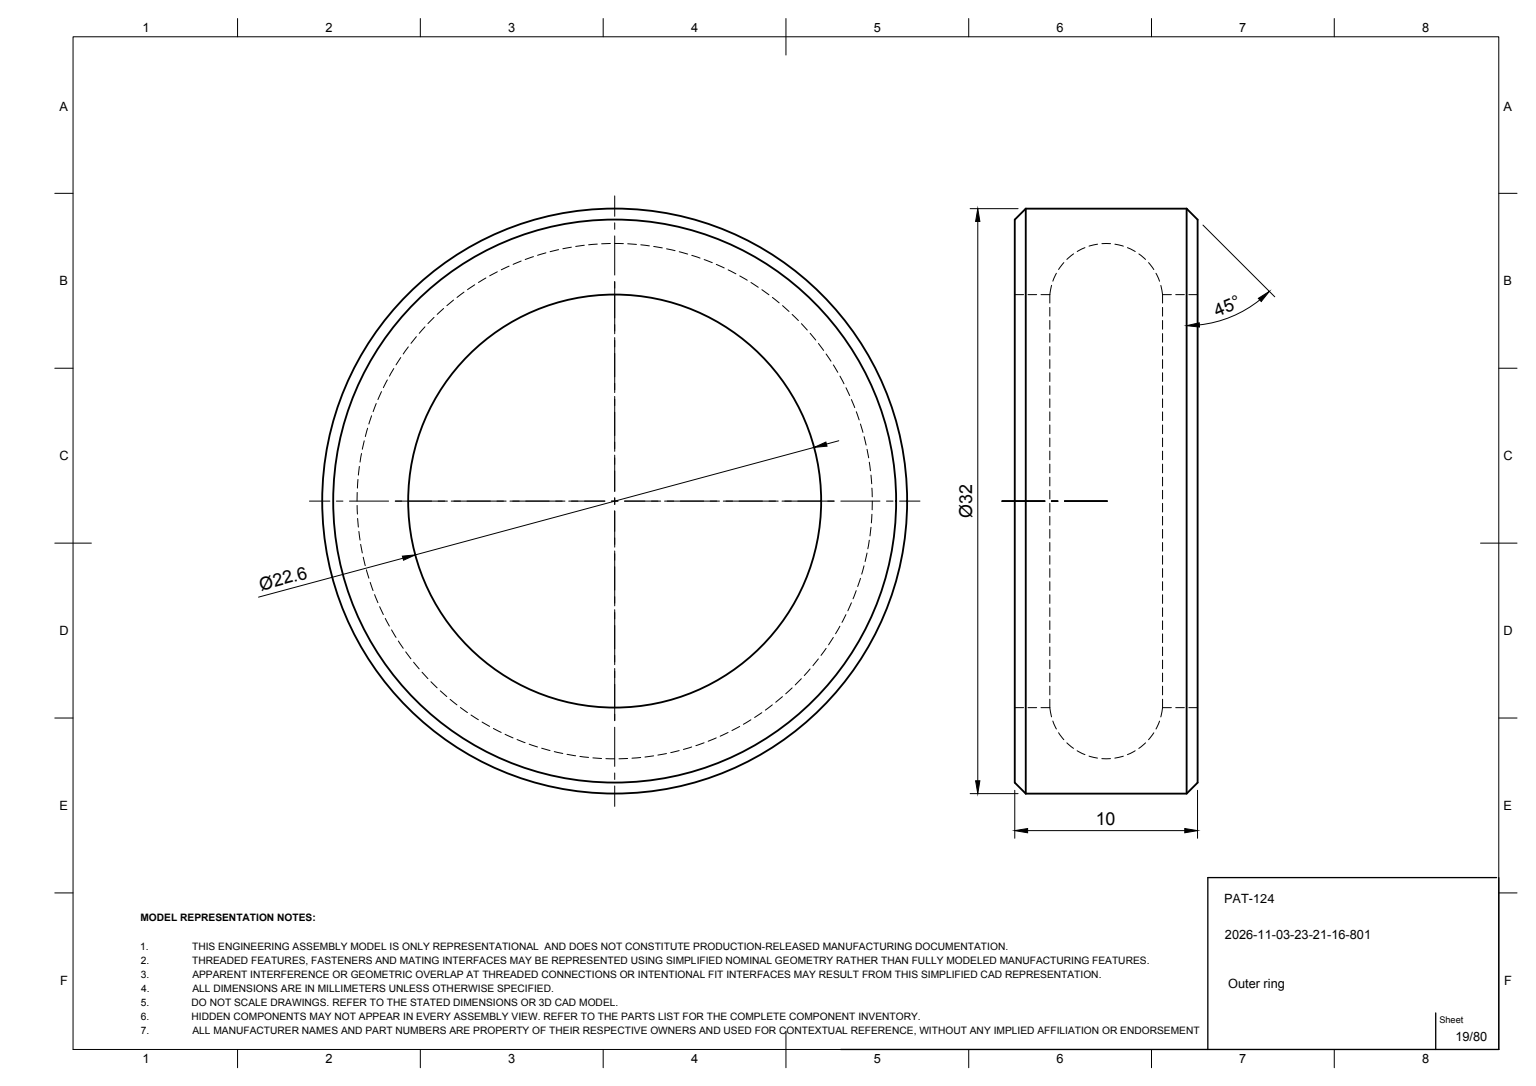
ISO-10303-21;
HEADER;
/* Generated by software containing ST-Developer
 * from STEP Tools, Inc. (www.steptools.com) 
 */

FILE_DESCRIPTION(
/* description */ ('XY cross-slide table'),
/* implementation_level */ '2;1');

FILE_NAME(
/* name */ 'Outer ring.step',
/* time_stamp */ '2026-10-28T03:22:46-07:00',
/* author */ (''),
/* organization */ (''),
/* preprocessor_version */ 'ST-DEVELOPER v20.2',
/* originating_system */ 'Autodesk Translation Framework v15.17.0.0',
/* authorisation */ '');

FILE_SCHEMA (('AUTOMOTIVE_DESIGN { 1 0 10303 214 3 1 1 }'));
ENDSEC;

DATA;
#10=MECHANICAL_DESIGN_GEOMETRIC_PRESENTATION_REPRESENTATION('',(#1682),#62984);
#1443=CONICAL_SURFACE('',#24318,1.57,0.785398163397449);
#1444=CONICAL_SURFACE('',#24322,1.57,0.785398163397449);
#1497=TOROIDAL_SURFACE('',#24307,1.1,0.309556);
#1516=SHAPE_REPRESENTATION_RELATIONSHIP('SRR','None',#63365,#1599);
#1599=ADVANCED_BREP_SHAPE_REPRESENTATION('',(#1795),#62902);
#1682=STYLED_ITEM('',(#63912),#1795);
#1795=MANIFOLD_SOLID_BREP('Body1',#22976);
#1985=FACE_BOUND('',#4439,.T.);
#1986=FACE_BOUND('',#4444,.T.);
#2383=PLANE('',#24315);
#2384=PLANE('',#24324);
#3024=FACE_OUTER_BOUND('',#4436,.T.);
#3025=FACE_OUTER_BOUND('',#4437,.T.);
#3026=FACE_OUTER_BOUND('',#4438,.T.);
#3027=FACE_OUTER_BOUND('',#4440,.T.);
#3028=FACE_OUTER_BOUND('',#4441,.T.);
#3029=FACE_OUTER_BOUND('',#4442,.T.);
#3030=FACE_OUTER_BOUND('',#4443,.T.);
#3031=FACE_OUTER_BOUND('',#4445,.T.);
#4436=EDGE_LOOP('',(#15586,#15587,#15588,#15589,#15590,#15591));
#4437=EDGE_LOOP('',(#15592,#15593,#15594,#15595,#15596));
#4438=EDGE_LOOP('',(#15597));
#4439=EDGE_LOOP('',(#15598));
#4440=EDGE_LOOP('',(#15599,#15600,#15601,#15602));
#4441=EDGE_LOOP('',(#15603,#15604,#15605,#15606));
#4442=EDGE_LOOP('',(#15607,#15608,#15609,#15610));
#4443=EDGE_LOOP('',(#15611));
#4444=EDGE_LOOP('',(#15612));
#4445=EDGE_LOOP('',(#15613,#15614,#15615,#15616,#15617));
#6112=LINE('',#33620,#7599);
#6113=LINE('',#33629,#7600);
#6114=LINE('',#33633,#7601);
#6115=LINE('',#33637,#7602);
#6116=LINE('',#33640,#7603);
#7599=VECTOR('',#27297,1.129765);
#7600=VECTOR('',#27308,1.57);
#7601=VECTOR('',#27313,1.6);
#7602=VECTOR('',#27318,1.57);
#7603=VECTOR('',#27323,1.129765);
#9015=CIRCLE('',#24308,1.129765);
#9016=CIRCLE('',#24309,1.129765);
#9017=CIRCLE('',#24310,0.309556);
#9018=CIRCLE('',#24311,1.129765);
#9019=CIRCLE('',#24312,1.129765);
#9020=CIRCLE('',#24314,1.129765);
#9021=CIRCLE('',#24316,1.54);
#9022=CIRCLE('',#24317,1.129765);
#9023=CIRCLE('',#24319,1.6);
#9024=CIRCLE('',#24321,1.6);
#9025=CIRCLE('',#24323,1.54);
#9997=VERTEX_POINT('',#33608);
#9998=VERTEX_POINT('',#33609);
#9999=VERTEX_POINT('',#33612);
#10000=VERTEX_POINT('',#33614);
#10001=VERTEX_POINT('',#33618);
#10002=VERTEX_POINT('',#33622);
#10003=VERTEX_POINT('',#33624);
#10004=VERTEX_POINT('',#33627);
#10005=VERTEX_POINT('',#33631);
#10006=VERTEX_POINT('',#33635);
#12177=EDGE_CURVE('',#9997,#9998,#9015,.T.);
#12178=EDGE_CURVE('',#9998,#9997,#9016,.T.);
#12179=EDGE_CURVE('',#9998,#9999,#9017,.T.);
#12180=EDGE_CURVE('',#10000,#9999,#9018,.T.);
#12181=EDGE_CURVE('',#9999,#10000,#9019,.T.);
#12182=EDGE_CURVE('',#10001,#10001,#9020,.T.);
#12183=EDGE_CURVE('',#10001,#10000,#6112,.T.);
#12184=EDGE_CURVE('',#10002,#10002,#9021,.T.);
#12185=EDGE_CURVE('',#10003,#10003,#9022,.T.);
#12186=EDGE_CURVE('',#10004,#10004,#9023,.T.);
#12187=EDGE_CURVE('',#10004,#10002,#6113,.T.);
#12188=EDGE_CURVE('',#10005,#10005,#9024,.T.);
#12189=EDGE_CURVE('',#10005,#10004,#6114,.T.);
#12190=EDGE_CURVE('',#10006,#10006,#9025,.T.);
#12191=EDGE_CURVE('',#10006,#10005,#6115,.T.);
#12192=EDGE_CURVE('',#9997,#10003,#6116,.T.);
#15586=ORIENTED_EDGE('',*,*,#12177,.F.);
#15587=ORIENTED_EDGE('',*,*,#12178,.F.);
#15588=ORIENTED_EDGE('',*,*,#12179,.T.);
#15589=ORIENTED_EDGE('',*,*,#12180,.F.);
#15590=ORIENTED_EDGE('',*,*,#12181,.F.);
#15591=ORIENTED_EDGE('',*,*,#12179,.F.);
#15592=ORIENTED_EDGE('',*,*,#12182,.T.);
#15593=ORIENTED_EDGE('',*,*,#12183,.T.);
#15594=ORIENTED_EDGE('',*,*,#12180,.T.);
#15595=ORIENTED_EDGE('',*,*,#12181,.T.);
#15596=ORIENTED_EDGE('',*,*,#12183,.F.);
#15597=ORIENTED_EDGE('',*,*,#12184,.F.);
#15598=ORIENTED_EDGE('',*,*,#12185,.T.);
#15599=ORIENTED_EDGE('',*,*,#12186,.F.);
#15600=ORIENTED_EDGE('',*,*,#12187,.T.);
#15601=ORIENTED_EDGE('',*,*,#12184,.T.);
#15602=ORIENTED_EDGE('',*,*,#12187,.F.);
#15603=ORIENTED_EDGE('',*,*,#12188,.F.);
#15604=ORIENTED_EDGE('',*,*,#12189,.T.);
#15605=ORIENTED_EDGE('',*,*,#12186,.T.);
#15606=ORIENTED_EDGE('',*,*,#12189,.F.);
#15607=ORIENTED_EDGE('',*,*,#12190,.F.);
#15608=ORIENTED_EDGE('',*,*,#12191,.T.);
#15609=ORIENTED_EDGE('',*,*,#12188,.T.);
#15610=ORIENTED_EDGE('',*,*,#12191,.F.);
#15611=ORIENTED_EDGE('',*,*,#12190,.T.);
#15612=ORIENTED_EDGE('',*,*,#12182,.F.);
#15613=ORIENTED_EDGE('',*,*,#12177,.T.);
#15614=ORIENTED_EDGE('',*,*,#12178,.T.);
#15615=ORIENTED_EDGE('',*,*,#12192,.T.);
#15616=ORIENTED_EDGE('',*,*,#12185,.F.);
#15617=ORIENTED_EDGE('',*,*,#12192,.F.);
#21105=CYLINDRICAL_SURFACE('',#24313,1.129765);
#21106=CYLINDRICAL_SURFACE('',#24320,1.6);
#21107=CYLINDRICAL_SURFACE('',#24325,1.129765);
#21805=ADVANCED_FACE('',(#3024),#1497,.F.);
#21806=ADVANCED_FACE('',(#3025),#21105,.F.);
#21807=ADVANCED_FACE('',(#3026,#1985),#2383,.T.);
#21808=ADVANCED_FACE('',(#3027),#1443,.T.);
#21809=ADVANCED_FACE('',(#3028),#21106,.T.);
#21810=ADVANCED_FACE('',(#3029),#1444,.T.);
#21811=ADVANCED_FACE('',(#3030,#1986),#2384,.T.);
#21812=ADVANCED_FACE('',(#3031),#21107,.F.);
#22976=CLOSED_SHELL('',(#21805,#21806,#21807,#21808,#21809,#21810,#21811,
#21812));
#24306=AXIS2_PLACEMENT_3D('',#33606,#27279,#27280);
#24307=AXIS2_PLACEMENT_3D('',#33607,#27281,#27282);
#24308=AXIS2_PLACEMENT_3D('',#33610,#27283,#27284);
#24309=AXIS2_PLACEMENT_3D('',#33611,#27285,#27286);
#24310=AXIS2_PLACEMENT_3D('',#33613,#27287,#27288);
#24311=AXIS2_PLACEMENT_3D('',#33615,#27289,#27290);
#24312=AXIS2_PLACEMENT_3D('',#33616,#27291,#27292);
#24313=AXIS2_PLACEMENT_3D('',#33617,#27293,#27294);
#24314=AXIS2_PLACEMENT_3D('',#33619,#27295,#27296);
#24315=AXIS2_PLACEMENT_3D('',#33621,#27298,#27299);
#24316=AXIS2_PLACEMENT_3D('',#33623,#27300,#27301);
#24317=AXIS2_PLACEMENT_3D('',#33625,#27302,#27303);
#24318=AXIS2_PLACEMENT_3D('',#33626,#27304,#27305);
#24319=AXIS2_PLACEMENT_3D('',#33628,#27306,#27307);
#24320=AXIS2_PLACEMENT_3D('',#33630,#27309,#27310);
#24321=AXIS2_PLACEMENT_3D('',#33632,#27311,#27312);
#24322=AXIS2_PLACEMENT_3D('',#33634,#27314,#27315);
#24323=AXIS2_PLACEMENT_3D('',#33636,#27316,#27317);
#24324=AXIS2_PLACEMENT_3D('',#33638,#27319,#27320);
#24325=AXIS2_PLACEMENT_3D('',#33639,#27321,#27322);
#27279=DIRECTION('axis',(0.,0.,1.));
#27280=DIRECTION('refdir',(1.,0.,0.));
#27281=DIRECTION('center_axis',(0.,-1.,0.));
#27282=DIRECTION('ref_axis',(0.,0.,-1.));
#27283=DIRECTION('center_axis',(0.,-1.,0.));
#27284=DIRECTION('ref_axis',(1.,0.,0.));
#27285=DIRECTION('center_axis',(0.,-1.,0.));
#27286=DIRECTION('ref_axis',(1.,0.,0.));
#27287=DIRECTION('center_axis',(1.,0.,1.22464679914735E-16));
#27288=DIRECTION('ref_axis',(-1.22464679914735E-16,0.,1.));
#27289=DIRECTION('center_axis',(0.,1.,0.));
#27290=DIRECTION('ref_axis',(1.,0.,0.));
#27291=DIRECTION('center_axis',(0.,1.,0.));
#27292=DIRECTION('ref_axis',(1.,0.,0.));
#27293=DIRECTION('center_axis',(0.,-1.,0.));
#27294=DIRECTION('ref_axis',(1.,0.,0.));
#27295=DIRECTION('center_axis',(0.,-1.,0.));
#27296=DIRECTION('ref_axis',(1.,0.,0.));
#27297=DIRECTION('',(0.,1.,0.));
#27298=DIRECTION('center_axis',(0.,1.,0.));
#27299=DIRECTION('ref_axis',(0.,0.,1.));
#27300=DIRECTION('center_axis',(0.,-1.,0.));
#27301=DIRECTION('ref_axis',(1.,0.,0.));
#27302=DIRECTION('center_axis',(0.,-1.,0.));
#27303=DIRECTION('ref_axis',(1.,0.,0.));
#27304=DIRECTION('center_axis',(0.,-1.,0.));
#27305=DIRECTION('ref_axis',(1.,0.,0.));
#27306=DIRECTION('center_axis',(0.,-1.,0.));
#27307=DIRECTION('ref_axis',(1.,0.,0.));
#27308=DIRECTION('',(0.707106781186548,0.707106781186547,8.65956056235494E-17));
#27309=DIRECTION('center_axis',(0.,-1.,0.));
#27310=DIRECTION('ref_axis',(1.,0.,0.));
#27311=DIRECTION('center_axis',(0.,-1.,0.));
#27312=DIRECTION('ref_axis',(1.,0.,0.));
#27313=DIRECTION('',(0.,1.,0.));
#27314=DIRECTION('center_axis',(0.,1.,0.));
#27315=DIRECTION('ref_axis',(1.,0.,0.));
#27316=DIRECTION('center_axis',(0.,-1.,0.));
#27317=DIRECTION('ref_axis',(1.,0.,0.));
#27318=DIRECTION('',(-0.707106781186548,0.707106781186547,-8.65956056235494E-17));
#27319=DIRECTION('center_axis',(0.,-1.,0.));
#27320=DIRECTION('ref_axis',(0.,0.,-1.));
#27321=DIRECTION('center_axis',(0.,-1.,0.));
#27322=DIRECTION('ref_axis',(1.,0.,0.));
#27323=DIRECTION('',(0.,1.,0.));
#33606=CARTESIAN_POINT('',(0.,0.,0.));
#33607=CARTESIAN_POINT('Origin',(0.,0.,0.));
#33608=CARTESIAN_POINT('',(-1.129765,0.308121667383195,-1.38356309103871E-16));
#33609=CARTESIAN_POINT('',(-1.38356309103871E-16,0.308121667383195,1.129765));
#33610=CARTESIAN_POINT('Origin',(0.,0.308121667383195,0.));
#33611=CARTESIAN_POINT('Origin',(0.,0.308121667383195,0.));
#33612=CARTESIAN_POINT('',(-1.38356309103871E-16,-0.308121667383195,1.129765));
#33613=CARTESIAN_POINT('Origin',(-1.34711147906209E-16,0.,1.1));
#33614=CARTESIAN_POINT('',(-1.129765,-0.308121667383195,1.38356309103871E-16));
#33615=CARTESIAN_POINT('Origin',(0.,-0.308121667383195,0.));
#33616=CARTESIAN_POINT('Origin',(0.,-0.308121667383195,0.));
#33617=CARTESIAN_POINT('Origin',(0.,0.,0.));
#33618=CARTESIAN_POINT('',(-1.129765,-0.5,-1.38356309103871E-16));
#33619=CARTESIAN_POINT('Origin',(0.,-0.5,0.));
#33620=CARTESIAN_POINT('',(-1.129765,0.,-1.38356309103871E-16));
#33621=CARTESIAN_POINT('Origin',(1.54,0.5,0.));
#33622=CARTESIAN_POINT('',(-1.54,0.5,-1.88595607068692E-16));
#33623=CARTESIAN_POINT('Origin',(0.,0.5,0.));
#33624=CARTESIAN_POINT('',(-1.129765,0.5,-1.38356309103871E-16));
#33625=CARTESIAN_POINT('Origin',(0.,0.5,0.));
#33626=CARTESIAN_POINT('Origin',(0.,0.47,0.));
#33627=CARTESIAN_POINT('',(-1.6,0.44,-1.95943487863577E-16));
#33628=CARTESIAN_POINT('Origin',(0.,0.44,0.));
#33629=CARTESIAN_POINT('',(-1.57,0.47,-1.92269547466134E-16));
#33630=CARTESIAN_POINT('Origin',(0.,0.,0.));
#33631=CARTESIAN_POINT('',(-1.6,-0.44,-1.95943487863577E-16));
#33632=CARTESIAN_POINT('Origin',(0.,-0.44,0.));
#33633=CARTESIAN_POINT('',(-1.6,0.,-1.95943487863577E-16));
#33634=CARTESIAN_POINT('Origin',(0.,-0.47,0.));
#33635=CARTESIAN_POINT('',(-1.54,-0.5,-1.88595607068692E-16));
#33636=CARTESIAN_POINT('Origin',(0.,-0.5,0.));
#33637=CARTESIAN_POINT('',(-1.57,-0.47,-1.92269547466134E-16));
#33638=CARTESIAN_POINT('Origin',(1.129765,-0.5,0.));
#33639=CARTESIAN_POINT('Origin',(0.,0.,0.));
#33640=CARTESIAN_POINT('',(-1.129765,0.,-1.38356309103871E-16));
#62803=UNCERTAINTY_MEASURE_WITH_UNIT(LENGTH_MEASURE(0.001),#62985,
'DISTANCE_ACCURACY_VALUE',
'Maximum model space distance between geometric entities at asserted c
onnectivities');
#62885=UNCERTAINTY_MEASURE_WITH_UNIT(LENGTH_MEASURE(0.001),#62985,
'DISTANCE_ACCURACY_VALUE',
'Maximum model space distance between geometric entities at asserted c
onnectivities');
#62902=(
GEOMETRIC_REPRESENTATION_CONTEXT(3)
GLOBAL_UNCERTAINTY_ASSIGNED_CONTEXT((#62803))
GLOBAL_UNIT_ASSIGNED_CONTEXT((#62985,#62987,#62988))
REPRESENTATION_CONTEXT('','3D')
);
#62984=(
GEOMETRIC_REPRESENTATION_CONTEXT(3)
GLOBAL_UNCERTAINTY_ASSIGNED_CONTEXT((#62885))
GLOBAL_UNIT_ASSIGNED_CONTEXT((#62985,#62987,#62988))
REPRESENTATION_CONTEXT('','3D')
);
#62985=(
LENGTH_UNIT()
NAMED_UNIT(*)
SI_UNIT(.CENTI.,.METRE.)
);
#62987=(
NAMED_UNIT(*)
PLANE_ANGLE_UNIT()
SI_UNIT($,.RADIAN.)
);
#62988=(
NAMED_UNIT(*)
SI_UNIT($,.STERADIAN.)
SOLID_ANGLE_UNIT()
);
#63005=SHAPE_DEFINITION_REPRESENTATION(#63103,#63365);
#63103=PRODUCT_DEFINITION_SHAPE('',$,#63464);
#63365=SHAPE_REPRESENTATION('',(#24306),#62902);
#63447=PRODUCT_DEFINITION_CONTEXT('part definition',#63743,'design');
#63464=PRODUCT_DEFINITION('Outer ring','Outer ring',#63562,#63447);
#63562=PRODUCT_DEFINITION_FORMATION('',$,#63761);
#63743=APPLICATION_CONTEXT(
'Core Data for Automotive Mechanical Design Process');
#63744=PRODUCT_CONTEXT('part definition',#63743,'mechanical');
#63761=PRODUCT('Outer ring','Outer ring','Outer ring',(#63744));
#63906=COLOUR_RGB('Grey',0.48,0.52,0.57);
#63907=FILL_AREA_STYLE_COLOUR('',#63906);
#63908=FILL_AREA_STYLE('',(#63907));
#63909=SURFACE_STYLE_FILL_AREA(#63908);
#63910=SURFACE_SIDE_STYLE('',(#63909));
#63911=SURFACE_STYLE_USAGE(.BOTH.,#63910);
#63912=PRESENTATION_STYLE_ASSIGNMENT((#63911));
ENDSEC;
END-ISO-10303-21;
